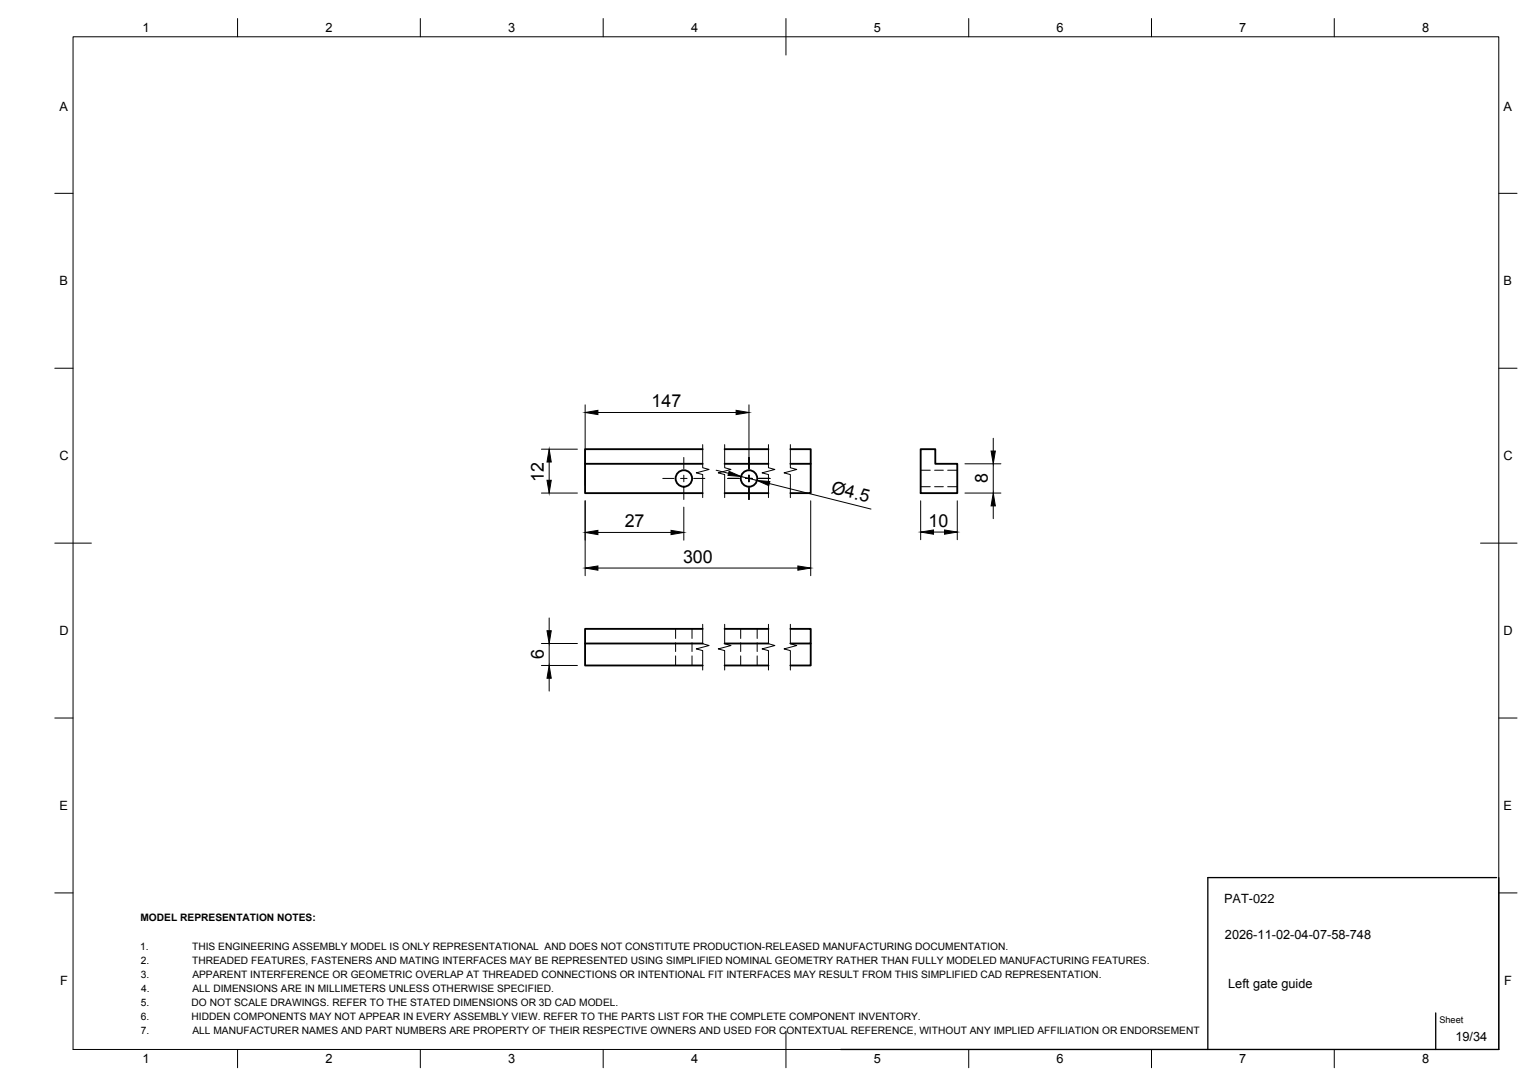
ISO-10303-21;
HEADER;
/* Generated by software containing ST-Developer
 * from STEP Tools, Inc. (www.steptools.com) 
 */

FILE_DESCRIPTION(
/* description */ ('Chute with adjustable gate'),
/* implementation_level */ '2;1');

FILE_NAME(
/* name */ 'Left gate guide.step',
/* time_stamp */ '2026-10-27T10:52:28-07:00',
/* author */ (''),
/* organization */ (''),
/* preprocessor_version */ 'ST-DEVELOPER v20.2',
/* originating_system */ 'Autodesk Translation Framework v15.17.0.0',
/* authorisation */ '');

FILE_SCHEMA (('AUTOMOTIVE_DESIGN { 1 0 10303 214 3 1 1 }'));
ENDSEC;

DATA;
#10=MECHANICAL_DESIGN_GEOMETRIC_PRESENTATION_REPRESENTATION('',(#428),#13094);
#364=SHAPE_REPRESENTATION_RELATIONSHIP('SRR','None',#13265,#396);
#396=ADVANCED_BREP_SHAPE_REPRESENTATION('',(#460),#13074);
#428=STYLED_ITEM('',(#13509),#460);
#460=MANIFOLD_SOLID_BREP('Body1',#7611);
#536=FACE_BOUND('',#1533,.T.);
#537=FACE_BOUND('',#1534,.T.);
#538=FACE_BOUND('',#1537,.T.);
#539=FACE_BOUND('',#1538,.T.);
#694=PLANE('',#8209);
#695=PLANE('',#8210);
#696=PLANE('',#8211);
#697=PLANE('',#8212);
#698=PLANE('',#8213);
#699=PLANE('',#8214);
#700=PLANE('',#8215);
#701=PLANE('',#8216);
#1050=FACE_OUTER_BOUND('',#1527,.T.);
#1051=FACE_OUTER_BOUND('',#1528,.T.);
#1052=FACE_OUTER_BOUND('',#1529,.T.);
#1053=FACE_OUTER_BOUND('',#1530,.T.);
#1054=FACE_OUTER_BOUND('',#1531,.T.);
#1055=FACE_OUTER_BOUND('',#1532,.T.);
#1056=FACE_OUTER_BOUND('',#1535,.T.);
#1057=FACE_OUTER_BOUND('',#1536,.T.);
#1058=FACE_OUTER_BOUND('',#1539,.T.);
#1059=FACE_OUTER_BOUND('',#1540,.T.);
#1527=EDGE_LOOP('',(#5786,#5787,#5788,#5789));
#1528=EDGE_LOOP('',(#5790,#5791,#5792,#5793));
#1529=EDGE_LOOP('',(#5794,#5795,#5796,#5797));
#1530=EDGE_LOOP('',(#5798,#5799,#5800,#5801));
#1531=EDGE_LOOP('',(#5802,#5803,#5804,#5805));
#1532=EDGE_LOOP('',(#5806,#5807,#5808,#5809));
#1533=EDGE_LOOP('',(#5810));
#1534=EDGE_LOOP('',(#5811));
#1535=EDGE_LOOP('',(#5812,#5813,#5814,#5815));
#1536=EDGE_LOOP('',(#5816,#5817,#5818,#5819));
#1537=EDGE_LOOP('',(#5820));
#1538=EDGE_LOOP('',(#5821));
#1539=EDGE_LOOP('',(#5822,#5823,#5824,#5825,#5826,#5827));
#1540=EDGE_LOOP('',(#5828,#5829,#5830,#5831,#5832,#5833));
#2096=LINE('',#11556,#2873);
#2097=LINE('',#11562,#2874);
#2098=LINE('',#11567,#2875);
#2099=LINE('',#11569,#2876);
#2100=LINE('',#11571,#2877);
#2101=LINE('',#11572,#2878);
#2102=LINE('',#11575,#2879);
#2103=LINE('',#11577,#2880);
#2104=LINE('',#11578,#2881);
#2105=LINE('',#11581,#2882);
#2106=LINE('',#11583,#2883);
#2107=LINE('',#11584,#2884);
#2108=LINE('',#11587,#2885);
#2109=LINE('',#11589,#2886);
#2110=LINE('',#11590,#2887);
#2111=LINE('',#11593,#2888);
#2112=LINE('',#11595,#2889);
#2113=LINE('',#11596,#2890);
#2114=LINE('',#11598,#2891);
#2115=LINE('',#11599,#2892);
#2873=VECTOR('',#9372,0.225000000000001);
#2874=VECTOR('',#9379,0.225000000000001);
#2875=VECTOR('',#9384,1.);
#2876=VECTOR('',#9385,1.);
#2877=VECTOR('',#9386,1.);
#2878=VECTOR('',#9387,1.);
#2879=VECTOR('',#9390,1.);
#2880=VECTOR('',#9391,1.);
#2881=VECTOR('',#9392,1.);
#2882=VECTOR('',#9395,1.);
#2883=VECTOR('',#9396,1.);
#2884=VECTOR('',#9397,1.);
#2885=VECTOR('',#9400,1.);
#2886=VECTOR('',#9401,1.);
#2887=VECTOR('',#9402,1.);
#2888=VECTOR('',#9405,1.);
#2889=VECTOR('',#9406,1.);
#2890=VECTOR('',#9407,1.);
#2891=VECTOR('',#9410,1.);
#2892=VECTOR('',#9411,1.);
#3478=CIRCLE('',#8204,0.225000000000001);
#3479=CIRCLE('',#8205,0.225000000000001);
#3480=CIRCLE('',#8207,0.225000000000001);
#3481=CIRCLE('',#8208,0.225000000000001);
#3793=VERTEX_POINT('',#11553);
#3794=VERTEX_POINT('',#11555);
#3795=VERTEX_POINT('',#11559);
#3796=VERTEX_POINT('',#11561);
#3797=VERTEX_POINT('',#11565);
#3798=VERTEX_POINT('',#11566);
#3799=VERTEX_POINT('',#11568);
#3800=VERTEX_POINT('',#11570);
#3801=VERTEX_POINT('',#11574);
#3802=VERTEX_POINT('',#11576);
#3803=VERTEX_POINT('',#11580);
#3804=VERTEX_POINT('',#11582);
#3805=VERTEX_POINT('',#11586);
#3806=VERTEX_POINT('',#11588);
#3807=VERTEX_POINT('',#11592);
#3808=VERTEX_POINT('',#11594);
#4526=EDGE_CURVE('',#3793,#3793,#3478,.T.);
#4527=EDGE_CURVE('',#3793,#3794,#2096,.T.);
#4528=EDGE_CURVE('',#3794,#3794,#3479,.T.);
#4529=EDGE_CURVE('',#3795,#3795,#3480,.T.);
#4530=EDGE_CURVE('',#3795,#3796,#2097,.T.);
#4531=EDGE_CURVE('',#3796,#3796,#3481,.T.);
#4532=EDGE_CURVE('',#3797,#3798,#2098,.T.);
#4533=EDGE_CURVE('',#3798,#3799,#2099,.T.);
#4534=EDGE_CURVE('',#3800,#3799,#2100,.T.);
#4535=EDGE_CURVE('',#3797,#3800,#2101,.T.);
#4536=EDGE_CURVE('',#3801,#3797,#2102,.T.);
#4537=EDGE_CURVE('',#3802,#3800,#2103,.T.);
#4538=EDGE_CURVE('',#3801,#3802,#2104,.T.);
#4539=EDGE_CURVE('',#3803,#3801,#2105,.T.);
#4540=EDGE_CURVE('',#3804,#3802,#2106,.T.);
#4541=EDGE_CURVE('',#3803,#3804,#2107,.T.);
#4542=EDGE_CURVE('',#3805,#3803,#2108,.T.);
#4543=EDGE_CURVE('',#3806,#3804,#2109,.T.);
#4544=EDGE_CURVE('',#3805,#3806,#2110,.T.);
#4545=EDGE_CURVE('',#3807,#3805,#2111,.T.);
#4546=EDGE_CURVE('',#3808,#3806,#2112,.T.);
#4547=EDGE_CURVE('',#3807,#3808,#2113,.T.);
#4548=EDGE_CURVE('',#3798,#3807,#2114,.T.);
#4549=EDGE_CURVE('',#3799,#3808,#2115,.T.);
#5786=ORIENTED_EDGE('',*,*,#4526,.F.);
#5787=ORIENTED_EDGE('',*,*,#4527,.T.);
#5788=ORIENTED_EDGE('',*,*,#4528,.F.);
#5789=ORIENTED_EDGE('',*,*,#4527,.F.);
#5790=ORIENTED_EDGE('',*,*,#4529,.F.);
#5791=ORIENTED_EDGE('',*,*,#4530,.T.);
#5792=ORIENTED_EDGE('',*,*,#4531,.F.);
#5793=ORIENTED_EDGE('',*,*,#4530,.F.);
#5794=ORIENTED_EDGE('',*,*,#4532,.T.);
#5795=ORIENTED_EDGE('',*,*,#4533,.T.);
#5796=ORIENTED_EDGE('',*,*,#4534,.F.);
#5797=ORIENTED_EDGE('',*,*,#4535,.F.);
#5798=ORIENTED_EDGE('',*,*,#4536,.T.);
#5799=ORIENTED_EDGE('',*,*,#4535,.T.);
#5800=ORIENTED_EDGE('',*,*,#4537,.F.);
#5801=ORIENTED_EDGE('',*,*,#4538,.F.);
#5802=ORIENTED_EDGE('',*,*,#4539,.T.);
#5803=ORIENTED_EDGE('',*,*,#4538,.T.);
#5804=ORIENTED_EDGE('',*,*,#4540,.F.);
#5805=ORIENTED_EDGE('',*,*,#4541,.F.);
#5806=ORIENTED_EDGE('',*,*,#4542,.T.);
#5807=ORIENTED_EDGE('',*,*,#4541,.T.);
#5808=ORIENTED_EDGE('',*,*,#4543,.F.);
#5809=ORIENTED_EDGE('',*,*,#4544,.F.);
#5810=ORIENTED_EDGE('',*,*,#4528,.T.);
#5811=ORIENTED_EDGE('',*,*,#4531,.T.);
#5812=ORIENTED_EDGE('',*,*,#4545,.T.);
#5813=ORIENTED_EDGE('',*,*,#4544,.T.);
#5814=ORIENTED_EDGE('',*,*,#4546,.F.);
#5815=ORIENTED_EDGE('',*,*,#4547,.F.);
#5816=ORIENTED_EDGE('',*,*,#4548,.T.);
#5817=ORIENTED_EDGE('',*,*,#4547,.T.);
#5818=ORIENTED_EDGE('',*,*,#4549,.F.);
#5819=ORIENTED_EDGE('',*,*,#4533,.F.);
#5820=ORIENTED_EDGE('',*,*,#4526,.T.);
#5821=ORIENTED_EDGE('',*,*,#4529,.T.);
#5822=ORIENTED_EDGE('',*,*,#4549,.T.);
#5823=ORIENTED_EDGE('',*,*,#4546,.T.);
#5824=ORIENTED_EDGE('',*,*,#4543,.T.);
#5825=ORIENTED_EDGE('',*,*,#4540,.T.);
#5826=ORIENTED_EDGE('',*,*,#4537,.T.);
#5827=ORIENTED_EDGE('',*,*,#4534,.T.);
#5828=ORIENTED_EDGE('',*,*,#4548,.F.);
#5829=ORIENTED_EDGE('',*,*,#4532,.F.);
#5830=ORIENTED_EDGE('',*,*,#4536,.F.);
#5831=ORIENTED_EDGE('',*,*,#4539,.F.);
#5832=ORIENTED_EDGE('',*,*,#4542,.F.);
#5833=ORIENTED_EDGE('',*,*,#4545,.F.);
#7138=CYLINDRICAL_SURFACE('',#8203,0.225000000000001);
#7139=CYLINDRICAL_SURFACE('',#8206,0.225000000000001);
#7318=ADVANCED_FACE('',(#1050),#7138,.F.);
#7319=ADVANCED_FACE('',(#1051),#7139,.F.);
#7320=ADVANCED_FACE('',(#1052),#694,.T.);
#7321=ADVANCED_FACE('',(#1053),#695,.T.);
#7322=ADVANCED_FACE('',(#1054),#696,.T.);
#7323=ADVANCED_FACE('',(#1055,#536,#537),#697,.T.);
#7324=ADVANCED_FACE('',(#1056),#698,.T.);
#7325=ADVANCED_FACE('',(#1057,#538,#539),#699,.T.);
#7326=ADVANCED_FACE('',(#1058),#700,.T.);
#7327=ADVANCED_FACE('',(#1059),#701,.F.);
#7611=CLOSED_SHELL('',(#7318,#7319,#7320,#7321,#7322,#7323,#7324,#7325,
#7326,#7327));
#8202=AXIS2_PLACEMENT_3D('',#11551,#9366,#9367);
#8203=AXIS2_PLACEMENT_3D('',#11552,#9368,#9369);
#8204=AXIS2_PLACEMENT_3D('',#11554,#9370,#9371);
#8205=AXIS2_PLACEMENT_3D('',#11557,#9373,#9374);
#8206=AXIS2_PLACEMENT_3D('',#11558,#9375,#9376);
#8207=AXIS2_PLACEMENT_3D('',#11560,#9377,#9378);
#8208=AXIS2_PLACEMENT_3D('',#11563,#9380,#9381);
#8209=AXIS2_PLACEMENT_3D('',#11564,#9382,#9383);
#8210=AXIS2_PLACEMENT_3D('',#11573,#9388,#9389);
#8211=AXIS2_PLACEMENT_3D('',#11579,#9393,#9394);
#8212=AXIS2_PLACEMENT_3D('',#11585,#9398,#9399);
#8213=AXIS2_PLACEMENT_3D('',#11591,#9403,#9404);
#8214=AXIS2_PLACEMENT_3D('',#11597,#9408,#9409);
#8215=AXIS2_PLACEMENT_3D('',#11600,#9412,#9413);
#8216=AXIS2_PLACEMENT_3D('',#11601,#9414,#9415);
#9366=DIRECTION('axis',(0.,0.,1.));
#9367=DIRECTION('refdir',(1.,0.,0.));
#9368=DIRECTION('center_axis',(1.,0.,0.));
#9369=DIRECTION('ref_axis',(0.,0.,-1.));
#9370=DIRECTION('center_axis',(1.,0.,0.));
#9371=DIRECTION('ref_axis',(0.,0.,-1.));
#9372=DIRECTION('',(1.,0.,0.));
#9373=DIRECTION('center_axis',(-1.,0.,0.));
#9374=DIRECTION('ref_axis',(0.,0.,-1.));
#9375=DIRECTION('center_axis',(1.,0.,0.));
#9376=DIRECTION('ref_axis',(0.,0.,-1.));
#9377=DIRECTION('center_axis',(1.,0.,0.));
#9378=DIRECTION('ref_axis',(0.,0.,-1.));
#9379=DIRECTION('',(1.,0.,0.));
#9380=DIRECTION('center_axis',(-1.,0.,0.));
#9381=DIRECTION('ref_axis',(0.,0.,-1.));
#9382=DIRECTION('center_axis',(0.,1.,0.));
#9383=DIRECTION('ref_axis',(-1.,0.,0.));
#9384=DIRECTION('',(-1.,0.,0.));
#9385=DIRECTION('',(0.,0.,1.));
#9386=DIRECTION('',(-1.,0.,0.));
#9387=DIRECTION('',(0.,0.,1.));
#9388=DIRECTION('center_axis',(1.,0.,0.));
#9389=DIRECTION('ref_axis',(0.,1.,0.));
#9390=DIRECTION('',(0.,1.,0.));
#9391=DIRECTION('',(0.,1.,0.));
#9392=DIRECTION('',(0.,0.,1.));
#9393=DIRECTION('center_axis',(0.,1.,0.));
#9394=DIRECTION('ref_axis',(-1.,0.,0.));
#9395=DIRECTION('',(-1.,0.,0.));
#9396=DIRECTION('',(-1.,0.,0.));
#9397=DIRECTION('',(0.,0.,1.));
#9398=DIRECTION('center_axis',(1.,0.,0.));
#9399=DIRECTION('ref_axis',(0.,1.,0.));
#9400=DIRECTION('',(0.,1.,0.));
#9401=DIRECTION('',(0.,1.,0.));
#9402=DIRECTION('',(0.,0.,1.));
#9403=DIRECTION('center_axis',(0.,-1.,0.));
#9404=DIRECTION('ref_axis',(1.,0.,0.));
#9405=DIRECTION('',(1.,0.,0.));
#9406=DIRECTION('',(1.,0.,0.));
#9407=DIRECTION('',(0.,0.,1.));
#9408=DIRECTION('center_axis',(-1.,0.,0.));
#9409=DIRECTION('ref_axis',(0.,-1.,0.));
#9410=DIRECTION('',(0.,-1.,0.));
#9411=DIRECTION('',(0.,-1.,0.));
#9412=DIRECTION('center_axis',(0.,0.,1.));
#9413=DIRECTION('ref_axis',(1.,0.,0.));
#9414=DIRECTION('center_axis',(0.,0.,1.));
#9415=DIRECTION('ref_axis',(1.,0.,0.));
#11551=CARTESIAN_POINT('',(0.,0.,0.));
#11552=CARTESIAN_POINT('Origin',(-2.1,-8.4,30.3));
#11553=CARTESIAN_POINT('',(-2.,-8.4,30.525));
#11554=CARTESIAN_POINT('Origin',(-2.,-8.4,30.3));
#11555=CARTESIAN_POINT('',(-1.,-8.4,30.525));
#11556=CARTESIAN_POINT('',(-2.1,-8.4,30.525));
#11557=CARTESIAN_POINT('Origin',(-1.,-8.4,30.3));
#11558=CARTESIAN_POINT('Origin',(-2.1,-8.4,18.3));
#11559=CARTESIAN_POINT('',(-2.,-8.4,18.525));
#11560=CARTESIAN_POINT('Origin',(-2.,-8.4,18.3));
#11561=CARTESIAN_POINT('',(-1.,-8.4,18.525));
#11562=CARTESIAN_POINT('',(-2.1,-8.4,18.525));
#11563=CARTESIAN_POINT('Origin',(-1.,-8.4,18.3));
#11564=CARTESIAN_POINT('Origin',(-1.6,-7.6,3.));
#11565=CARTESIAN_POINT('',(-1.6,-7.6,3.));
#11566=CARTESIAN_POINT('',(-2.,-7.6,3.));
#11567=CARTESIAN_POINT('',(-1.6,-7.6,3.));
#11568=CARTESIAN_POINT('',(-2.,-7.6,33.));
#11569=CARTESIAN_POINT('',(-2.,-7.6,3.));
#11570=CARTESIAN_POINT('',(-1.6,-7.6,33.));
#11571=CARTESIAN_POINT('',(-1.6,-7.6,33.));
#11572=CARTESIAN_POINT('',(-1.6,-7.6,3.));
#11573=CARTESIAN_POINT('Origin',(-1.6,-8.,3.));
#11574=CARTESIAN_POINT('',(-1.6,-8.,3.));
#11575=CARTESIAN_POINT('',(-1.6,-8.,3.));
#11576=CARTESIAN_POINT('',(-1.6,-8.,33.));
#11577=CARTESIAN_POINT('',(-1.6,-8.,33.));
#11578=CARTESIAN_POINT('',(-1.6,-8.,3.));
#11579=CARTESIAN_POINT('Origin',(-1.,-8.,3.));
#11580=CARTESIAN_POINT('',(-1.,-8.,3.));
#11581=CARTESIAN_POINT('',(-1.,-8.,3.));
#11582=CARTESIAN_POINT('',(-1.,-8.,33.));
#11583=CARTESIAN_POINT('',(-1.,-8.,33.));
#11584=CARTESIAN_POINT('',(-1.,-8.,3.));
#11585=CARTESIAN_POINT('Origin',(-1.,-8.8,3.));
#11586=CARTESIAN_POINT('',(-1.,-8.8,3.));
#11587=CARTESIAN_POINT('',(-1.,-8.8,3.));
#11588=CARTESIAN_POINT('',(-1.,-8.8,33.));
#11589=CARTESIAN_POINT('',(-1.,-8.8,33.));
#11590=CARTESIAN_POINT('',(-1.,-8.8,3.));
#11591=CARTESIAN_POINT('Origin',(-2.,-8.8,3.));
#11592=CARTESIAN_POINT('',(-2.,-8.8,3.));
#11593=CARTESIAN_POINT('',(-2.,-8.8,3.));
#11594=CARTESIAN_POINT('',(-2.,-8.8,33.));
#11595=CARTESIAN_POINT('',(-2.,-8.8,33.));
#11596=CARTESIAN_POINT('',(-2.,-8.8,3.));
#11597=CARTESIAN_POINT('Origin',(-2.,-7.6,3.));
#11598=CARTESIAN_POINT('',(-2.,-7.6,3.));
#11599=CARTESIAN_POINT('',(-2.,-7.6,33.));
#11600=CARTESIAN_POINT('Origin',(-1.5,-8.2,33.));
#11601=CARTESIAN_POINT('Origin',(-1.5,-8.2,3.));
#13037=UNCERTAINTY_MEASURE_WITH_UNIT(LENGTH_MEASURE(0.001),#13095,
'DISTANCE_ACCURACY_VALUE',
'Maximum model space distance between geometric entities at asserted c
onnectivities');
#13057=UNCERTAINTY_MEASURE_WITH_UNIT(LENGTH_MEASURE(0.001),#13095,
'DISTANCE_ACCURACY_VALUE',
'Maximum model space distance between geometric entities at asserted c
onnectivities');
#13074=(
GEOMETRIC_REPRESENTATION_CONTEXT(3)
GLOBAL_UNCERTAINTY_ASSIGNED_CONTEXT((#13037))
GLOBAL_UNIT_ASSIGNED_CONTEXT((#13095,#13097,#13098))
REPRESENTATION_CONTEXT('','3D')
);
#13094=(
GEOMETRIC_REPRESENTATION_CONTEXT(3)
GLOBAL_UNCERTAINTY_ASSIGNED_CONTEXT((#13057))
GLOBAL_UNIT_ASSIGNED_CONTEXT((#13095,#13097,#13098))
REPRESENTATION_CONTEXT('','3D')
);
#13095=(
LENGTH_UNIT()
NAMED_UNIT(*)
SI_UNIT(.CENTI.,.METRE.)
);
#13097=(
NAMED_UNIT(*)
PLANE_ANGLE_UNIT()
SI_UNIT($,.RADIAN.)
);
#13098=(
NAMED_UNIT(*)
SI_UNIT($,.STERADIAN.)
SOLID_ANGLE_UNIT()
);
#13115=SHAPE_DEFINITION_REPRESENTATION(#13151,#13265);
#13151=PRODUCT_DEFINITION_SHAPE('',$,#13302);
#13265=SHAPE_REPRESENTATION('',(#8202),#13074);
#13285=PRODUCT_DEFINITION_CONTEXT('part definition',#13395,'design');
#13302=PRODUCT_DEFINITION('Left gate guide','Left gate guide',#13338,#13285);
#13338=PRODUCT_DEFINITION_FORMATION('',$,#13413);
#13395=APPLICATION_CONTEXT(
'Core Data for Automotive Mechanical Design Process');
#13396=PRODUCT_CONTEXT('part definition',#13395,'mechanical');
#13413=PRODUCT('Left gate guide','Left gate guide','Left gate guide',(#13396));
#13503=COLOUR_RGB('Off White',0.89,0.88,0.83);
#13504=FILL_AREA_STYLE_COLOUR('',#13503);
#13505=FILL_AREA_STYLE('',(#13504));
#13506=SURFACE_STYLE_FILL_AREA(#13505);
#13507=SURFACE_SIDE_STYLE('',(#13506));
#13508=SURFACE_STYLE_USAGE(.BOTH.,#13507);
#13509=PRESENTATION_STYLE_ASSIGNMENT((#13508));
ENDSEC;
END-ISO-10303-21;
